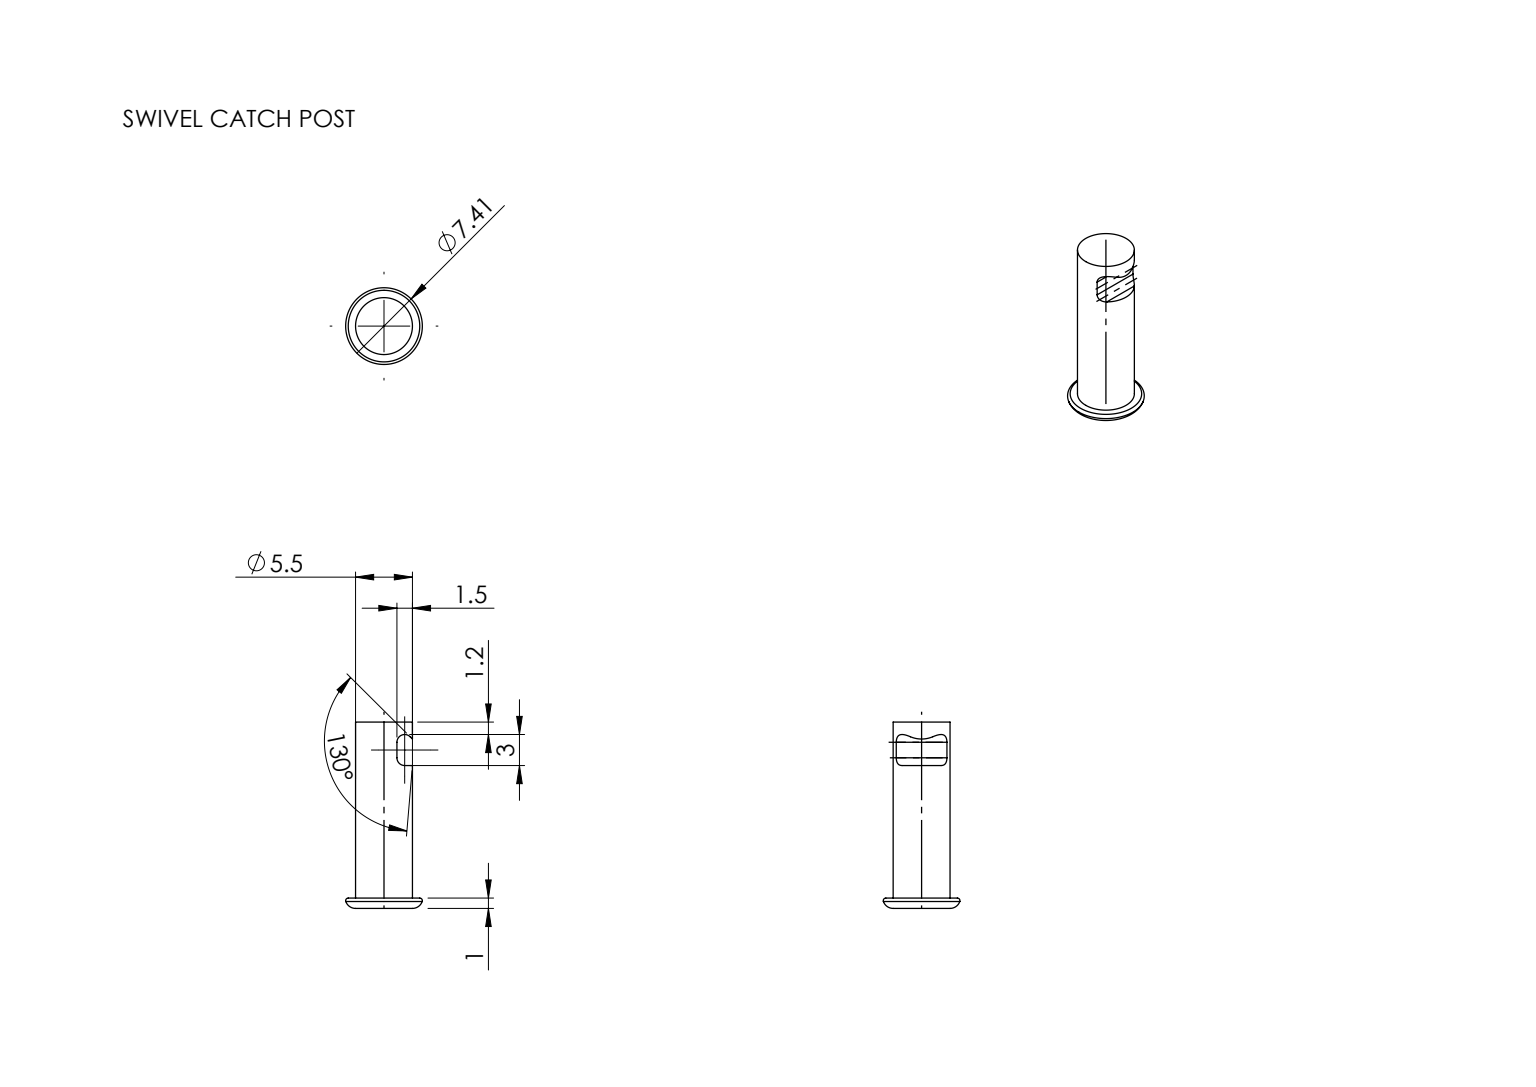
ISO-10303-21;
HEADER;
FILE_DESCRIPTION (('STEP AP214'),
    '1' );
FILE_NAME ('Swivel Catch Post.step',
    '2026-09-30T04:43:20',
    ( '' ),
    ( '' ),
    'SwSTEP 2.0',
    'SolidWorks 2026',
    '' );
FILE_SCHEMA (( 'AUTOMOTIVE_DESIGN' ));
ENDSEC;

DATA;
#106=EDGE_CURVE ( 'NONE', #30303, #19164, #12974, .T. ) ;
#210=LINE ( 'NONE', #17557, #51006 ) ;
#446=ADVANCED_FACE ( 'NONE', ( #32795 ), #44037, .T. ) ;
#717=FACE_OUTER_BOUND ( 'NONE', #44823, .T. ) ;
#818=DIRECTION ( 'NONE',  ( 0.000000000000000000, 1.000000000000000000, 0.000000000000000000 ) ) ;
#927=CARTESIAN_POINT ( 'NONE',  ( -56.75000000000000711, 6.050000000000001599, 2.449489742783185875 ) ) ;
#976=DIRECTION ( 'NONE',  ( 0.000000000000000000, -1.000000000000000000, 0.000000000000000000 ) ) ;
#1009=CIRCLE ( 'NONE', #16413, 2.750000000000001776 ) ;
#1234=CYLINDRICAL_SURFACE ( 'NONE', #12104, 0.7500000000000006661 ) ;
#1569=ORIENTED_EDGE ( 'NONE', *, *, #18264, .F. ) ;
#1965=ORIENTED_EDGE ( 'NONE', *, *, #43779, .F. ) ;
#2198=ORIENTED_EDGE ( 'NONE', *, *, #35348, .F. ) ;
#2411=MANIFOLD_SOLID_BREP ( 'Fillet2', #42168 ) ;
#2610=AXIS2_PLACEMENT_3D ( 'NONE', #34638, #13373, #3697 ) ;
#2848=CARTESIAN_POINT ( 'NONE',  ( -55.47117325737978888, 6.581829179614757663, 1.080525476705103127 ) ) ;
#3278=( NAMED_UNIT ( * ) PLANE_ANGLE_UNIT ( ) SI_UNIT ( $, .RADIAN. ) );
#3473=ADVANCED_FACE ( 'NONE', ( #50960, #8114 ), #12651, .T. ) ;
#3535=VERTEX_POINT ( 'NONE', #55238 ) ;
#3551=( LENGTH_UNIT ( ) NAMED_UNIT ( * ) SI_UNIT ( .MILLI., .METRE. ) );
#3578=CARTESIAN_POINT ( 'NONE',  ( -58.00000000000000711, -9.999999999999998224, 7.102951435054649637E-15 ) ) ;
#3629=CARTESIAN_POINT ( 'NONE',  ( -56.65747392845349850, 6.423369595003239674, -2.400381607668001571 ) ) ;
#3697=DIRECTION ( 'NONE',  ( 1.000000000000000000, 0.000000000000000000, 0.000000000000000000 ) ) ;
#3987=CIRCLE ( 'NONE', #7590, 3.692809041582069352 ) ;
#4028=EDGE_LOOP ( 'NONE', ( #26060, #54634 ) ) ;
#4049=ORIENTED_EDGE ( 'NONE', *, *, #41228, .F. ) ;
#4164=CIRCLE ( 'NONE', #6875, 1.000000000000000000 ) ;
#4191=DIRECTION ( 'NONE',  ( -0.000000000000000000, -0.000000000000000000, 1.000000000000000000 ) ) ;
#4239=FACE_OUTER_BOUND ( 'NONE', #21147, .T. ) ;
#4283=ORIENTED_EDGE ( 'NONE', *, *, #8142, .T. ) ;
#4454=EDGE_CURVE ( 'NONE', #51315, #45422, #36769, .T. ) ;
#4485=CARTESIAN_POINT ( 'NONE',  ( -55.79576865894325977, 6.773981352271770007, -1.647106450292881163 ) ) ;
#4595=DIRECTION ( 'NONE',  ( 0.000000000000000000, 0.000000000000000000, 1.000000000000000000 ) ) ;
#4651=ORIENTED_EDGE ( 'NONE', *, *, #24419, .F. ) ;
#4656=PRODUCT ( 'Swivel Catch Post', 'Swivel Catch Post', '', ( #13009 ) ) ;
#4836=CIRCLE ( 'NONE', #42891, 3.457106781186553235 ) ;
#4927=EDGE_LOOP ( 'NONE', ( #9077, #36170 ) ) ;
#5049=ADVANCED_FACE ( 'NONE', ( #50607 ), #46482, .T. ) ;
#5155=DIRECTION ( 'NONE',  ( -0.000000000000000000, -0.000000000000000000, 1.000000000000000000 ) ) ;
#5423=EDGE_CURVE ( 'NONE', #11807, #36151, #4836, .T. ) ;
#5489=EDGE_LOOP ( 'NONE', ( #39206, #54488 ) ) ;
#5657=TOROIDAL_SURFACE ( 'NONE', #31069, 3.457106781186553235, 0.2500000000000000000 ) ;
#5758=AXIS2_PLACEMENT_3D ( 'NONE', #44985, #31062, #44404 ) ;
#5852=CIRCLE ( 'NONE', #10392, 2.750000000000001776 ) ;
#6089=PRODUCT_DEFINITION_SHAPE ( 'NONE', 'NONE',  #46837 ) ;
#6098=AXIS2_PLACEMENT_3D ( 'NONE', #52656, #26020, #51820 ) ;
#6342=EDGE_CURVE ( 'NONE', #47897, #8966, #3987, .T. ) ;
#6579=CARTESIAN_POINT ( 'NONE',  ( -55.97617513261492661, 6.813462753686547302, 1.872163189751866907 ) ) ;
#6606=EDGE_LOOP ( 'NONE', ( #41022, #15281, #4651, #28201 ) ) ;
#6772=DIRECTION ( 'NONE',  ( 0.000000000000000000, 1.000000000000000000, 0.000000000000000000 ) ) ;
#6829=CARTESIAN_POINT ( 'NONE',  ( -58.00000000000000711, -8.999999999999998224, 2.750000000000013323 ) ) ;
#6875=AXIS2_PLACEMENT_3D ( 'NONE', #10848, #23077, #23368 ) ;
#6928=CARTESIAN_POINT ( 'NONE',  ( -56.00000000000000711, 3.800000000000001599, 1.887458608817694561 ) ) ;
#7213=CARTESIAN_POINT ( 'NONE',  ( -58.00000000000000711, -9.000000000000000000, 7.102951435054649637E-15 ) ) ;
#7257=CARTESIAN_POINT ( 'NONE',  ( -55.47117325737978888, 6.581829179614757663, -1.080525476705088916 ) ) ;
#7453=EDGE_CURVE ( 'NONE', #8966, #47897, #15484, .T. ) ;
#7541=DIRECTION ( 'NONE',  ( 0.000000000000000000, 1.000000000000000000, 0.000000000000000000 ) ) ;
#7590=AXIS2_PLACEMENT_3D ( 'NONE', #8285, #25599, #12827 ) ;
#7684=CARTESIAN_POINT ( 'NONE',  ( -55.47117325737978888, 6.581829179614757663, -1.080525476705088916 ) ) ;
#7794=VECTOR ( 'NONE', #30262, 1000.000000000000000 ) ;
#8114=FACE_OUTER_BOUND ( 'NONE', #6606, .T. ) ;
#8142=EDGE_CURVE ( 'NONE', #45422, #51315, #1009, .T. ) ;
#8210=ORIENTED_EDGE ( 'NONE', *, *, #43779, .T. ) ;
#8223=ORIENTED_EDGE ( 'NONE', *, *, #14640, .T. ) ;
#8264=ORIENTED_EDGE ( 'NONE', *, *, #40320, .F. ) ;
#8285=CARTESIAN_POINT ( 'NONE',  ( -58.00000000000000711, -9.333333333333333925, 7.102951435054649637E-15 ) ) ;
#8429=DIRECTION ( 'NONE',  ( 0.000000000000000000, 1.000000000000000000, 0.000000000000000000 ) ) ;
#8475=DIRECTION ( 'NONE',  ( 0.000000000000000000, 0.000000000000000000, -1.000000000000000000 ) ) ;
#8786=DIRECTION ( 'NONE',  ( -0.000000000000000000, -0.000000000000000000, 1.000000000000000000 ) ) ;
#8966=VERTEX_POINT ( 'NONE', #28731 ) ;
#9077=ORIENTED_EDGE ( 'NONE', *, *, #4454, .F. ) ;
#9245=ORIENTED_EDGE ( 'NONE', *, *, #7453, .T. ) ;
#9495=DIRECTION ( 'NONE',  ( -0.000000000000000000, -0.000000000000000000, 1.000000000000000000 ) ) ;
#9731=AXIS2_PLACEMENT_3D ( 'NONE', #16881, #48351, #13173 ) ;
#9733=CARTESIAN_POINT ( 'NONE',  ( -56.32517369257367079, 3.868430646962533359, -2.183859404458766917 ) ) ;
#9746=APPLICATION_CONTEXT ( 'automotive_design' ) ;
#9865=EDGE_CURVE ( 'NONE', #3535, #28311, #56017, .T. ) ;
#9936=CARTESIAN_POINT ( 'NONE',  ( -58.00000000000000711, -9.000000000000000000, -3.457106781186546129 ) ) ;
#9965=CARTESIAN_POINT ( 'NONE',  ( -58.00000000000000711, -9.000000000000000000, 2.750000000000008438 ) ) ;
#10333=DIRECTION ( 'NONE',  ( -1.000000000000000000, 0.000000000000000000, -0.000000000000000000 ) ) ;
#10392=AXIS2_PLACEMENT_3D ( 'NONE', #34327, #12733, #8475 ) ;
#10736=FACE_OUTER_BOUND ( 'NONE', #5489, .T. ) ;
#10786=ADVANCED_FACE ( 'NONE', ( #10736 ), #24058, .F. ) ;
#10848=CARTESIAN_POINT ( 'NONE',  ( -58.00000000000000711, -8.999999999999998224, -2.749999999999999556 ) ) ;
#10855=CARTESIAN_POINT ( 'NONE',  ( -24.28770178542860947, -24.42559627614718565, -2.749999999999994671 ) ) ;
#10888=CARTESIAN_POINT ( 'NONE',  ( -56.40932156468398517, 3.913516004366899725, 2.245148959471634065 ) ) ;
#10909=DIRECTION ( 'NONE',  ( 0.000000000000000000, -1.000000000000000000, 0.000000000000000000 ) ) ;
#10925=EDGE_CURVE ( 'NONE', #36151, #11807, #55038, .T. ) ;
#11019=ORIENTED_EDGE ( 'NONE', *, *, #7453, .F. ) ;
#11426=ADVANCED_FACE ( 'NONE', ( #56060 ), #17711, .T. ) ;
#11522=DIRECTION ( 'NONE',  ( 0.000000000000000000, -1.000000000000000000, 0.000000000000000000 ) ) ;
#11576=DIRECTION ( 'NONE',  ( -0.000000000000000000, 1.000000000000000000, -0.000000000000000000 ) ) ;
#11607=EDGE_CURVE ( 'NONE', #45422, #39433, #35883, .T. ) ;
#11689=ORIENTED_EDGE ( 'NONE', *, *, #26993, .T. ) ;
#11777=ORIENTED_EDGE ( 'NONE', *, *, #41228, .T. ) ;
#11807=VERTEX_POINT ( 'NONE', #9936 ) ;
#11982=CARTESIAN_POINT ( 'NONE',  ( -56.75000000000000711, -9.000000000000000000, -2.449489742783172108 ) ) ;
#12104=AXIS2_PLACEMENT_3D ( 'NONE', #44676, #9495, #18868 ) ;
#12280=ORIENTED_EDGE ( 'NONE', *, *, #21641, .F. ) ;
#12377=FILL_AREA_STYLE ('',( #29957 ) ) ;
#12476=DIRECTION ( 'NONE',  ( 1.000000000000000000, 0.000000000000000000, 0.000000000000000000 ) ) ;
#12488=AXIS2_PLACEMENT_3D ( 'NONE', #3578, #25186, #41901 ) ;
#12651=CYLINDRICAL_SURFACE ( 'NONE', #41209, 2.750000000000001776 ) ;
#12705=ADVANCED_FACE ( 'NONE', ( #52110 ), #55979, .T. ) ;
#12717=CARTESIAN_POINT ( 'NONE',  ( -56.40927410319390134, 6.683688692736960313, -2.245073662639579304 ) ) ;
#12726=SHAPE_DEFINITION_REPRESENTATION ( #6089, #55389 ) ;
#12733=DIRECTION ( 'NONE',  ( -0.000000000000000000, 1.000000000000000000, -0.000000000000000000 ) ) ;
#12827=DIRECTION ( 'NONE',  ( 0.000000000000000000, 0.000000000000000000, 1.000000000000000000 ) ) ;
#12917=AXIS2_PLACEMENT_3D ( 'NONE', #7213, #10909, #24263 ) ;
#12974=LINE ( 'NONE', #47317, #16801 ) ;
#13009=PRODUCT_CONTEXT ( 'NONE', #9746, 'mechanical' ) ;
#13173=DIRECTION ( 'NONE',  ( 0.000000000000000000, -0.000000000000000000, -1.000000000000000000 ) ) ;
#13373=DIRECTION ( 'NONE',  ( 0.000000000000000000, 0.000000000000000000, 1.000000000000000000 ) ) ;
#13398=CARTESIAN_POINT ( 'NONE',  ( -56.75000000000000711, 6.050000000000001599, -2.749999999999994671 ) ) ;
#13741=FACE_OUTER_BOUND ( 'NONE', #52868, .T. ) ;
#13747=EDGE_LOOP ( 'NONE', ( #25210, #8223, #11019, #4049 ) ) ;
#13765=CARTESIAN_POINT ( 'NONE',  ( -58.00000000000000711, -9.250000000000000000, 7.102951435054649637E-15 ) ) ;
#13893=DIRECTION ( 'NONE',  ( 0.000000000000000000, 1.000000000000000000, 0.000000000000000000 ) ) ;
#14023=CARTESIAN_POINT ( 'NONE',  ( -58.00000000000000711, -9.000000000000000000, 7.102951435054649637E-15 ) ) ;
#14277=CARTESIAN_POINT ( 'NONE',  ( -56.75000000000000711, 4.550000000000001599, -2.449489742783172108 ) ) ;
#14309=CARTESIAN_POINT ( 'NONE',  ( -58.00000000000000711, -9.000000000000000000, -2.749999999999994671 ) ) ;
#14387=EDGE_CURVE ( 'NONE', #8966, #28311, #4164, .T. ) ;
#14529=CARTESIAN_POINT ( 'NONE',  ( -56.75000000000000711, 4.436543092327784876, -2.449489742783172996 ) ) ;
#14559=DIRECTION ( 'NONE',  ( 0.7091055728196409280, -0.7051023234936394379, 0.000000000000000000 ) ) ;
#14640=EDGE_CURVE ( 'NONE', #36151, #47897, #36794, .T. ) ;
#14755=CIRCLE ( 'NONE', #43758, 2.750000000000001776 ) ;
#14829=CARTESIAN_POINT ( 'NONE',  ( -56.40853634832227925, 6.684187361877747868, 2.244562702769390405 ) ) ;
#14841=FACE_OUTER_BOUND ( 'NONE', #33369, .T. ) ;
#15281=ORIENTED_EDGE ( 'NONE', *, *, #11607, .T. ) ;
#15484=CIRCLE ( 'NONE', #38148, 3.692809041582069352 ) ;
#15630=CARTESIAN_POINT ( 'NONE',  ( -58.00000000000000711, -9.999999999999998224, 7.102951435054649637E-15 ) ) ;
#15739=CIRCLE ( 'NONE', #47489, 1.000000000000000000 ) ;
#15804=DIRECTION ( 'NONE',  ( 0.000000000000000000, 0.000000000000000000, -1.000000000000000000 ) ) ;
#15899=AXIS2_PLACEMENT_3D ( 'NONE', #36805, #11522, #41039 ) ;
#15965=AXIS2_PLACEMENT_3D ( 'NONE', #30563, #52950, #39053 ) ;
#16203=CARTESIAN_POINT ( 'NONE',  ( -55.17209868701984732, 6.284443032133043339, -0.3805810627426228776 ) ) ;
#16235=COLOUR_RGB ( '', 0.09019608, 0.27058824, 0.51372549) ;
#16258=APPLICATION_CONTEXT ( 'automotive_design' ) ;
#16298=CARTESIAN_POINT ( 'NONE',  ( -58.00000000000000711, 8.000000000000000000, 7.102951435054649637E-15 ) ) ;
#16413=AXIS2_PLACEMENT_3D ( 'NONE', #49665, #6772, #45126 ) ;
#16474=SURFACE_STYLE_FILL_AREA ( #34949 ) ;
#16801=VECTOR ( 'NONE', #4191, 1000.000000000000000 ) ;
#16831=ADVANCED_FACE ( 'NONE', ( #27358 ), #36184, .F. ) ;
#16834=CARTESIAN_POINT ( 'NONE',  ( -58.00000000000000711, 8.000000000000000000, 7.102951435054649637E-15 ) ) ;
#16881=CARTESIAN_POINT ( 'NONE',  ( -58.00000000000000711, -9.999999999999998224, 7.102951435054649637E-15 ) ) ;
#17063=( NAMED_UNIT ( * ) SI_UNIT ( $, .STERADIAN. ) SOLID_ANGLE_UNIT ( ) );
#17413=DIRECTION ( 'NONE',  ( 0.000000000000000000, 0.000000000000000000, 1.000000000000000000 ) ) ;
#17534=CARTESIAN_POINT ( 'NONE',  ( -56.60431429388330571, 6.503145704592061982, -2.370631253071207922 ) ) ;
#17557=CARTESIAN_POINT ( 'NONE',  ( -56.00000000000000711, 3.800000000000001599, -2.749999999999994671 ) ) ;
#17640=DIRECTION ( 'NONE',  ( 0.000000000000000000, 1.000000000000000000, 0.000000000000000000 ) ) ;
#17664=DIRECTION ( 'NONE',  ( 0.000000000000000000, -1.000000000000000000, 0.000000000000000000 ) ) ;
#17711=PLANE ( 'NONE',  #9731 ) ;
#18264=EDGE_CURVE ( 'NONE', #48789, #29854, #42161, .T. ) ;
#18503=CARTESIAN_POINT ( 'NONE',  ( -56.15823370927599001, 3.811598478745688023, -2.045038383219965894 ) ) ;
#18868=DIRECTION ( 'NONE',  ( 1.000000000000000000, 0.000000000000000000, 0.000000000000000000 ) ) ;
#19164=VERTEX_POINT ( 'NONE', #31350 ) ;
#19352=CARTESIAN_POINT ( 'NONE',  ( -55.84725198092744591, 6.793269954351565332, 1.721684726214605998 ) ) ;
#19364=DIRECTION ( 'NONE',  ( -0.7051023234936394379, -0.7091055728196409280, 0.000000000000000000 ) ) ;
#20049=CARTESIAN_POINT ( 'NONE',  ( -58.00000000000000711, -9.000000000000000000, 7.102951435054649637E-15 ) ) ;
#20178=CARTESIAN_POINT ( 'NONE',  ( -55.54283117668188652, 6.653082554758466216, 1.248231344413326394 ) ) ;
#20257=FACE_OUTER_BOUND ( 'NONE', #4028, .T. ) ;
#20315=CARTESIAN_POINT ( 'NONE',  ( -58.00000000000000711, 8.000000000000000000, 7.102951435054649637E-15 ) ) ;
#20494=VERTEX_POINT ( 'NONE', #39393 ) ;
#20778=STYLED_ITEM ( 'NONE', ( #47425 ), #49640 ) ;
#20796=FACE_OUTER_BOUND ( 'NONE', #42057, .T. ) ;
#20913=VERTEX_POINT ( 'NONE', #35839 ) ;
#21012=SHAPE_REPRESENTATION_RELATIONSHIP ( 'NONE' , 'NONE' ,  #55389, #49640 ) ;
#21116=LINE ( 'NONE', #35057, #30207 ) ;
#21147=EDGE_LOOP ( 'NONE', ( #31251, #25114, #24414, #22015 ) ) ;
#21202=ORIENTED_EDGE ( 'NONE', *, *, #14387, .F. ) ;
#21641=EDGE_CURVE ( 'NONE', #40359, #30303, #40783, .T. ) ;
#21701=DIRECTION ( 'NONE',  ( 0.000000000000000000, 1.000000000000000000, 0.000000000000000000 ) ) ;
#21726=PRODUCT_DEFINITION_FORMATION_WITH_SPECIFIED_SOURCE ( 'ANY', '', #4656, .NOT_KNOWN. ) ;
#21740=CYLINDRICAL_SURFACE ( 'NONE', #15965, 2.750000000000001776 ) ;
#21794=CARTESIAN_POINT ( 'NONE',  ( -56.75000000000000711, 6.050000000000001599, -2.449489742783172108 ) ) ;
#21847=EDGE_CURVE ( 'NONE', #39433, #20494, #14755, .T. ) ;
#22015=ORIENTED_EDGE ( 'NONE', *, *, #23716, .F. ) ;
#22053=VECTOR ( 'NONE', #17640, 1000.000000000000000 ) ;
#22431=EDGE_LOOP ( 'NONE', ( #30912, #42795, #39124, #36013, #33556, #12280, #2198, #1569 ) ) ;
#23015=ORIENTED_EDGE ( 'NONE', *, *, #31360, .T. ) ;
#23077=DIRECTION ( 'NONE',  ( -1.000000000000000000, -0.000000000000000000, -0.000000000000000000 ) ) ;
#23368=DIRECTION ( 'NONE',  ( 0.000000000000000000, 0.000000000000000000, 1.000000000000000000 ) ) ;
#23492=ADVANCED_FACE ( 'NONE', ( #14841 ), #53721, .T. ) ;
#23716=EDGE_CURVE ( 'NONE', #40359, #47613, #48273, .T. ) ;
#23946=CARTESIAN_POINT ( 'NONE',  ( -56.07727432805427981, 3.800000000000001155, 1.969340487120371019 ) ) ;
#24058=PLANE ( 'NONE',  #46848 ) ;
#24195=CARTESIAN_POINT ( 'NONE',  ( -56.65661634607675978, 6.425189153618619642, 2.399912804366261643 ) ) ;
#24263=DIRECTION ( 'NONE',  ( 0.000000000000000000, -0.000000000000000000, -1.000000000000000000 ) ) ;
#24409=DIRECTION ( 'NONE',  ( 1.000000000000000000, 0.000000000000000000, -1.224646799147353207E-16 ) ) ;
#24414=ORIENTED_EDGE ( 'NONE', *, *, #39666, .T. ) ;
#24419=EDGE_CURVE ( 'NONE', #20494, #39433, #42009, .T. ) ;
#24686=EDGE_LOOP ( 'NONE', ( #39980, #48644, #11777, #45574 ) ) ;
#25090=CARTESIAN_POINT ( 'NONE',  ( -56.75000000000001421, 4.436683557093994423, 2.449489742783185875 ) ) ;
#25114=ORIENTED_EDGE ( 'NONE', *, *, #106, .T. ) ;
#25186=DIRECTION ( 'NONE',  ( 0.000000000000000000, -1.000000000000000000, 0.000000000000000000 ) ) ;
#25210=ORIENTED_EDGE ( 'NONE', *, *, #10925, .F. ) ;
#25232=CARTESIAN_POINT ( 'NONE',  ( -56.75000000000001421, 6.148917331397711017, -2.449489742783171664 ) ) ;
#25420=DIRECTION ( 'NONE',  ( 0.000000000000000000, 0.000000000000000000, 1.000000000000000000 ) ) ;
#25488=CARTESIAN_POINT ( 'NONE',  ( -55.63255288014424593, 6.714018351055213607, -1.412117554830255362 ) ) ;
#25599=DIRECTION ( 'NONE',  ( 0.000000000000000000, -1.000000000000000000, 0.000000000000000000 ) ) ;
#25865=( NAMED_UNIT ( * ) PLANE_ANGLE_UNIT ( ) SI_UNIT ( $, .RADIAN. ) );
#25936=AXIS2_PLACEMENT_3D ( 'NONE', #34392, #30421, #51973 ) ;
#26020=DIRECTION ( 'NONE',  ( 0.000000000000000000, -1.000000000000000000, 0.000000000000000000 ) ) ;
#26060=ORIENTED_EDGE ( 'NONE', *, *, #5423, .T. ) ;
#26080=CARTESIAN_POINT ( 'NONE',  ( -56.26447305843585411, 6.756484714774108724, -2.135113782577493513 ) ) ;
#26136=CARTESIAN_POINT ( 'NONE',  ( -55.17209868701984732, 6.284443032133044227, 0.3805810627426376991 ) ) ;
#26396=( LENGTH_UNIT ( ) NAMED_UNIT ( * ) SI_UNIT ( .MILLI., .METRE. ) );
#26610=VECTOR ( 'NONE', #34165, 1000.000000000000000 ) ;
#26938=CARTESIAN_POINT ( 'NONE',  ( -56.75000000000000711, 6.050000000000001599, -2.449489742783172108 ) ) ;
#26993=EDGE_CURVE ( 'NONE', #50717, #20913, #34858, .T. ) ;
#27040=CARTESIAN_POINT ( 'NONE',  ( -56.40918267430362221, 3.913378331250040087, -2.245061400351528569 ) ) ;
#27358=FACE_OUTER_BOUND ( 'NONE', #28823, .T. ) ;
#27706=CIRCLE ( 'NONE', #47728, 2.750000000000006217 ) ;
#28043=CARTESIAN_POINT ( 'NONE',  ( 0.000000000000000000, 3.800000000000002043, -2.749999999999994671 ) ) ;
#28156=CARTESIAN_POINT ( 'NONE',  ( -56.60439204777216560, 6.503221467314357795, 2.370703063681847134 ) ) ;
#28201=ORIENTED_EDGE ( 'NONE', *, *, #47935, .F. ) ;
#28203=CARTESIAN_POINT ( 'NONE',  ( -56.32449333261072155, 3.868143273367939727, 2.183322036886178097 ) ) ;
#28311=VERTEX_POINT ( 'NONE', #36142 ) ;
#28504=PLANE ( 'NONE',  #12917 ) ;
#28731=CARTESIAN_POINT ( 'NONE',  ( -58.00000000000000711, -9.333333333333333925, -3.692809041582062246 ) ) ;
#28823=EDGE_LOOP ( 'NONE', ( #32458, #1965, #52851, #40119 ) ) ;
#29107=PRODUCT_DEFINITION_CONTEXT ( 'detailed design', #16258, 'design' ) ;
#29112=CARTESIAN_POINT ( 'NONE',  ( -58.00000000000000711, -9.000000000000000000, 7.102951435054649637E-15 ) ) ;
#29396=( NAMED_UNIT ( * ) SI_UNIT ( $, .STERADIAN. ) SOLID_ANGLE_UNIT ( ) );
#29573=( NAMED_UNIT ( * ) SI_UNIT ( $, .STERADIAN. ) SOLID_ANGLE_UNIT ( ) );
#29854=VERTEX_POINT ( 'NONE', #44099 ) ;
#29957=FILL_AREA_STYLE_COLOUR ( '', #48271 ) ;
#30036=CARTESIAN_POINT ( 'NONE',  ( -56.19068569781688893, 6.778861748851165103, -2.073212483771301073 ) ) ;
#30183=EDGE_LOOP ( 'NONE', ( #23015, #48028 ) ) ;
#30207=VECTOR ( 'NONE', #47527, 1000.000000000000000 ) ;
#30262=DIRECTION ( 'NONE',  ( -0.000000000000000000, -0.000000000000000000, 1.000000000000000000 ) ) ;
#30303=VERTEX_POINT ( 'NONE', #7257 ) ;
#30404=SURFACE_STYLE_USAGE ( .BOTH. , #51121 ) ;
#30421=DIRECTION ( 'NONE',  ( 1.000000000000000000, 0.000000000000000000, -1.224646799147353207E-16 ) ) ;
#30563=CARTESIAN_POINT ( 'NONE',  ( -58.00000000000000711, -9.000000000000000000, 7.102951435054649637E-15 ) ) ;
#30912=ORIENTED_EDGE ( 'NONE', *, *, #48807, .F. ) ;
#31062=DIRECTION ( 'NONE',  ( -1.000000000000000000, -0.000000000000000000, -0.000000000000000000 ) ) ;
#31069=AXIS2_PLACEMENT_3D ( 'NONE', #13765, #976, #31932 ) ;
#31251=ORIENTED_EDGE ( 'NONE', *, *, #21641, .T. ) ;
#31294=CARTESIAN_POINT ( 'NONE',  ( -56.07732056155856526, 3.800000000000001155, -1.969389477338281624 ) ) ;
#31350=CARTESIAN_POINT ( 'NONE',  ( -55.47117325737978888, 6.581829179614757663, 1.080525476705103127 ) ) ;
#31360=EDGE_CURVE ( 'NONE', #28311, #3535, #27706, .T. ) ;
#31932=DIRECTION ( 'NONE',  ( 0.000000000000000000, 0.000000000000000000, -1.000000000000000000 ) ) ;
#31960=STYLED_ITEM ( 'NONE', ( #37636 ), #2411 ) ;
#32458=ORIENTED_EDGE ( 'NONE', *, *, #47523, .T. ) ;
#32493=CARTESIAN_POINT ( 'NONE',  ( -56.63016842841614817, 4.129031330634377994, 2.385144069838411873 ) ) ;
#32510=FACE_BOUND ( 'NONE', #4927, .T. ) ;
#32795=FACE_OUTER_BOUND ( 'NONE', #53183, .T. ) ;
#32979=CARTESIAN_POINT ( 'NONE',  ( -56.47915852223218280, 6.634043282999704694, 2.292377755077263934 ) ) ;
#33369=EDGE_LOOP ( 'NONE', ( #42457, #56083 ) ) ;
#33556=ORIENTED_EDGE ( 'NONE', *, *, #36953, .T. ) ;
#33666=( BOUNDED_CURVE ( )  B_SPLINE_CURVE ( 3, ( #42336, #26136, #16203, #7684 ),
 .UNSPECIFIED., .F., .F. ) 
 B_SPLINE_CURVE_WITH_KNOTS ( ( 4, 4 ),
 ( 2.737789607505189515, 3.545395699674396717 ),
 .UNSPECIFIED. ) 
 CURVE ( )  GEOMETRIC_REPRESENTATION_ITEM ( )  RATIONAL_B_SPLINE_CURVE ( ( 1.000000000000000000, 0.9463822406352063732, 0.9463822406352063732, 1.000000000000000000 ) ) 
 REPRESENTATION_ITEM ( '' )  );
#33805=( NAMED_UNIT ( * ) PLANE_ANGLE_UNIT ( ) SI_UNIT ( $, .RADIAN. ) );
#34165=DIRECTION ( 'NONE',  ( 0.000000000000000000, 1.000000000000000000, 0.000000000000000000 ) ) ;
#34327=CARTESIAN_POINT ( 'NONE',  ( -58.00000000000000711, 3.800000000000002931, 7.102951435054649637E-15 ) ) ;
#34340=EDGE_CURVE ( 'NONE', #47897, #3535, #15739, .T. ) ;
#34392=CARTESIAN_POINT ( 'NONE',  ( -58.00000000000000711, -9.250000000000000000, 3.457106781186559896 ) ) ;
#34508=LINE ( 'NONE', #51821, #7794 ) ;
#34534=ORIENTED_EDGE ( 'NONE', *, *, #6342, .T. ) ;
#34638=CARTESIAN_POINT ( 'NONE',  ( 0.000000000000000000, 0.000000000000000000, 0.000000000000000000 ) ) ;
#34693=CARTESIAN_POINT ( 'NONE',  ( -58.00000000000000711, -9.333333333333333925, 7.102951435054649637E-15 ) ) ;
#34858=B_SPLINE_CURVE_WITH_KNOTS ( 'NONE', 3,
 ( #54327, #25090, #37278, #32493, #49795, #10888, #28203, #45512, #23946, #6928 ),
 .UNSPECIFIED., .F., .F.,
 ( 4, 2, 2, 2, 4 ),
 ( 0.000000000000000000, 0.0003349897808261797561, 0.0006699795616523595123, 0.001004969342478539323, 0.001339959123304719025 ),
 .UNSPECIFIED. ) ;
#34949=FILL_AREA_STYLE ('',( #56227 ) ) ;
#35057=CARTESIAN_POINT ( 'NONE',  ( -56.75000000000000711, -9.000000000000000000, 2.449489742783185875 ) ) ;
#35308=MECHANICAL_DESIGN_GEOMETRIC_PRESENTATION_REPRESENTATION('',(#20778),#52518);
#35343=ADVANCED_FACE ( 'NONE', ( #20796 ), #55718, .T. ) ;
#35348=EDGE_CURVE ( 'NONE', #29854, #40359, #55426, .T. ) ;
#35362=FACE_OUTER_BOUND ( 'NONE', #13747, .T. ) ;
#35660=AXIS2_PLACEMENT_3D ( 'NONE', #16834, #818, #48227 ) ;
#35738=AXIS2_PLACEMENT_3D ( 'NONE', #50314, #41530, #40952 ) ;
#35839=CARTESIAN_POINT ( 'NONE',  ( -56.00000000000000711, 3.800000000000001599, 1.887458608817694561 ) ) ;
#35846=CARTESIAN_POINT ( 'NONE',  ( -56.56312404709360919, 4.044422194259722936, -2.346569400431943730 ) ) ;
#35883=LINE ( 'NONE', #14309, #54960 ) ;
#36013=ORIENTED_EDGE ( 'NONE', *, *, #39666, .F. ) ;
#36142=CARTESIAN_POINT ( 'NONE',  ( -58.00000000000000711, -9.999999999999998224, -2.749999999999999556 ) ) ;
#36151=VERTEX_POINT ( 'NONE', #52097 ) ;
#36170=ORIENTED_EDGE ( 'NONE', *, *, #8142, .F. ) ;
#36184=PLANE ( 'NONE',  #54068 ) ;
#36608=AXIS2_PLACEMENT_3D ( 'NONE', #55322, #47090, #12476 ) ;
#36691=CARTESIAN_POINT ( 'NONE',  ( -56.75000000000000711, 6.050000000000001599, 2.449489742783185875 ) ) ;
#36769=CIRCLE ( 'NONE', #42226, 2.750000000000001776 ) ;
#36794=CIRCLE ( 'NONE', #25936, 0.2499999999999997780 ) ;
#36805=CARTESIAN_POINT ( 'NONE',  ( -58.00000000000000711, -8.999999999999998224, 7.102951435054649637E-15 ) ) ;
#36953=EDGE_CURVE ( 'NONE', #19164, #30303, #33666, .T. ) ;
#37092=UNCERTAINTY_MEASURE_WITH_UNIT (LENGTH_MEASURE( 1.000000000000000082E-05 ), #3551, 'distance_accuracy_value', 'NONE');
#37227=CARTESIAN_POINT ( 'NONE',  ( -56.73047118268372202, 6.245764598936942136, 2.439786402985463898 ) ) ;
#37278=CARTESIAN_POINT ( 'NONE',  ( -56.72378334990722237, 4.325356880459150233, 2.436518382942996830 ) ) ;
#37384=DIRECTION ( 'NONE',  ( 0.000000000000000000, 0.000000000000000000, -1.000000000000000000 ) ) ;
#37515=CARTESIAN_POINT ( 'NONE',  ( -56.19049806081029175, 6.779003593249485426, 2.073111974254101320 ) ) ;
#37636=PRESENTATION_STYLE_ASSIGNMENT (( #42463 ) ) ;
#37650=DIRECTION ( 'NONE',  ( 0.000000000000000000, 1.000000000000000000, 0.000000000000000000 ) ) ;
#38148=AXIS2_PLACEMENT_3D ( 'NONE', #34693, #17664, #4595 ) ;
#38259=CARTESIAN_POINT ( 'NONE',  ( -56.48048524421252381, 6.632812770515467804, -2.293230480183058528 ) ) ;
#38371=LINE ( 'NONE', #43224, #22053 ) ;
#38417=AXIS2_PLACEMENT_3D ( 'NONE', #16298, #21701, #17413 ) ;
#38910=( GEOMETRIC_REPRESENTATION_CONTEXT ( 3 ) GLOBAL_UNCERTAINTY_ASSIGNED_CONTEXT ( ( #51263 ) ) GLOBAL_UNIT_ASSIGNED_CONTEXT ( ( #26396, #33805, #17063 ) ) REPRESENTATION_CONTEXT ( 'NONE', 'WORKASPACE' ) );
#39053=DIRECTION ( 'NONE',  ( 0.000000000000000000, 0.000000000000000000, 1.000000000000000000 ) ) ;
#39110=CARTESIAN_POINT ( 'NONE',  ( -55.47117325737978888, 6.581829179614757663, -1.080525476705088916 ) ) ;
#39124=ORIENTED_EDGE ( 'NONE', *, *, #47523, .F. ) ;
#39206=ORIENTED_EDGE ( 'NONE', *, *, #40320, .T. ) ;
#39291=ADVANCED_FACE ( 'NONE', ( #35362 ), #5657, .T. ) ;
#39334=ADVANCED_FACE ( 'NONE', ( #20257, #32510 ), #28504, .F. ) ;
#39393=CARTESIAN_POINT ( 'NONE',  ( -58.00000000000000711, 8.000000000000000000, 2.750000000000008438 ) ) ;
#39433=VERTEX_POINT ( 'NONE', #45532 ) ;
#39595=ORIENTED_EDGE ( 'NONE', *, *, #34340, .T. ) ;
#39666=EDGE_CURVE ( 'NONE', #19164, #47613, #50163, .T. ) ;
#39980=ORIENTED_EDGE ( 'NONE', *, *, #14640, .F. ) ;
#40119=ORIENTED_EDGE ( 'NONE', *, *, #23716, .T. ) ;
#40191=ORIENTED_EDGE ( 'NONE', *, *, #18264, .T. ) ;
#40320=EDGE_CURVE ( 'NONE', #48789, #20913, #210, .T. ) ;
#40359=VERTEX_POINT ( 'NONE', #26938 ) ;
#40519=ORIENTED_EDGE ( 'NONE', *, *, #47935, .T. ) ;
#40664=CARTESIAN_POINT ( 'NONE',  ( -56.62967144059850000, 4.128180327486781209, -2.384865143139781374 ) ) ;
#40710=DIRECTION ( 'NONE',  ( 0.000000000000000000, 0.000000000000000000, 1.000000000000000000 ) ) ;
#40783=B_SPLINE_CURVE_WITH_KNOTS ( 'NONE', 3,
 ( #21794, #25232, #42538, #3629, #17534, #38259, #12717, #26080, #30036, #55583, #51346, #43389, #4485, #25488, #42796, #39110 ),
 .UNSPECIFIED., .F., .F.,
 ( 4, 2, 2, 2, 2, 2, 2, 4 ),
 ( 0.000000000000000000, 0.0002924226556627319796, 0.0005848453113254639592, 0.0008772679669881960473, 0.001169690622650927918, 0.001462113278313660440, 0.001754535933976393179, 0.002339381245301844995 ),
 .UNSPECIFIED. ) ;
#40952=DIRECTION ( 'NONE',  ( 0.000000000000000000, 0.000000000000000000, -1.000000000000000000 ) ) ;
#41022=ORIENTED_EDGE ( 'NONE', *, *, #4454, .T. ) ;
#41039=DIRECTION ( 'NONE',  ( 0.000000000000000000, 0.000000000000000000, -1.000000000000000000 ) ) ;
#41194=ADVANCED_FACE ( 'NONE', ( #13741 ), #1234, .F. ) ;
#41209=AXIS2_PLACEMENT_3D ( 'NONE', #29112, #37650, #25420 ) ;
#41221=CARTESIAN_POINT ( 'NONE',  ( -55.63114022126601554, 6.713117369705148718, 1.409618983554703719 ) ) ;
#41228=EDGE_CURVE ( 'NONE', #11807, #8966, #48386, .T. ) ;
#41511=CARTESIAN_POINT ( 'NONE',  ( -56.75000000000001421, 6.149180203093333574, 2.449489742783260038 ) ) ;
#41530=DIRECTION ( 'NONE',  ( 0.000000000000000000, -1.000000000000000000, 0.000000000000000000 ) ) ;
#41749=DIRECTION ( 'NONE',  ( 0.000000000000000000, 0.000000000000000000, -1.000000000000000000 ) ) ;
#41901=DIRECTION ( 'NONE',  ( 0.000000000000000000, 0.000000000000000000, -1.000000000000000000 ) ) ;
#42009=CIRCLE ( 'NONE', #38417, 2.750000000000001776 ) ;
#42057=EDGE_LOOP ( 'NONE', ( #54737, #55252 ) ) ;
#42147=CARTESIAN_POINT ( 'NONE',  ( -56.75000000000000711, 4.550000000000001599, 2.449489742783185875 ) ) ;
#42161=B_SPLINE_CURVE_WITH_KNOTS ( 'NONE', 3,
 ( #48622, #31294, #18503, #9733, #27040, #35846, #40664, #53169, #14529, #14277 ),
 .UNSPECIFIED., .F., .F.,
 ( 4, 2, 2, 2, 4 ),
 ( 0.000000000000000000, 0.0003339141718491685099, 0.0006678283436983370198, 0.001001742515547505638, 0.001335656687396674040 ),
 .UNSPECIFIED. ) ;
#42168=CLOSED_SHELL ( 'NONE', ( #39291, #12705, #3473, #43879, #35343, #10786, #41194, #16831, #48753, #23492, #11426, #39334, #446, #5049 ) ) ;
#42172=SURFACE_STYLE_FILL_AREA ( #12377 ) ;
#42188=DIRECTION ( 'NONE',  ( 0.000000000000000000, 0.000000000000000000, 1.000000000000000000 ) ) ;
#42226=AXIS2_PLACEMENT_3D ( 'NONE', #14023, #8429, #40710 ) ;
#42336=CARTESIAN_POINT ( 'NONE',  ( -55.47117325737978888, 6.581829179614757663, 1.080525476705103127 ) ) ;
#42457=ORIENTED_EDGE ( 'NONE', *, *, #106, .F. ) ;
#42463=SURFACE_STYLE_USAGE ( .BOTH. , #46714 ) ;
#42538=CARTESIAN_POINT ( 'NONE',  ( -56.73021393513262467, 6.246123507023290777, -2.439641667270313619 ) ) ;
#42795=ORIENTED_EDGE ( 'NONE', *, *, #26993, .F. ) ;
#42796=CARTESIAN_POINT ( 'NONE',  ( -55.54282512360118318, 6.653076535853754692, -1.248217177980195380 ) ) ;
#42891=AXIS2_PLACEMENT_3D ( 'NONE', #51317, #11576, #37384 ) ;
#43224=CARTESIAN_POINT ( 'NONE',  ( -58.00000000000000711, -9.000000000000000000, 2.750000000000008438 ) ) ;
#43281=ORIENTED_EDGE ( 'NONE', *, *, #11607, .F. ) ;
#43389=CARTESIAN_POINT ( 'NONE',  ( -55.85443948382626900, 6.788488266608555755, -1.722920386167723583 ) ) ;
#43475=ORIENTED_EDGE ( 'NONE', *, *, #34340, .F. ) ;
#43736=MECHANICAL_DESIGN_GEOMETRIC_PRESENTATION_REPRESENTATION('',(#31960),#50984);
#43758=AXIS2_PLACEMENT_3D ( 'NONE', #20315, #7541, #42188 ) ;
#43779=EDGE_CURVE ( 'NONE', #29854, #50717, #34508, .T. ) ;
#43879=ADVANCED_FACE ( 'NONE', ( #717 ), #21740, .T. ) ;
#44037=TOROIDAL_SURFACE ( 'NONE', #15899, 2.750000000000006217, 1.000000000000000000 ) ;
#44099=CARTESIAN_POINT ( 'NONE',  ( -56.75000000000000711, 4.550000000000001599, -2.449489742783172108 ) ) ;
#44404=DIRECTION ( 'NONE',  ( 0.000000000000000000, 0.000000000000000000, 1.000000000000000000 ) ) ;
#44676=CARTESIAN_POINT ( 'NONE',  ( -56.00000000000000711, 4.550000000000001599, -2.749999999999994671 ) ) ;
#44735=ORIENTED_EDGE ( 'NONE', *, *, #14387, .T. ) ;
#44823=EDGE_LOOP ( 'NONE', ( #43281, #4283, #40519, #50145 ) ) ;
#44985=CARTESIAN_POINT ( 'NONE',  ( -58.00000000000000711, -9.250000000000000000, -3.457106781186546129 ) ) ;
#45126=DIRECTION ( 'NONE',  ( 0.000000000000000000, 0.000000000000000000, 1.000000000000000000 ) ) ;
#45280=ORIENTED_EDGE ( 'NONE', *, *, #31360, .F. ) ;
#45347=DIRECTION ( 'NONE',  ( 0.000000000000000000, -0.000000000000000000, -1.000000000000000000 ) ) ;
#45422=VERTEX_POINT ( 'NONE', #55068 ) ;
#45512=CARTESIAN_POINT ( 'NONE',  ( -56.15805904048855979, 3.811595058059581209, 2.044864594757502818 ) ) ;
#45532=CARTESIAN_POINT ( 'NONE',  ( -58.00000000000000711, 8.000000000000000000, -2.749999999999994671 ) ) ;
#45574=ORIENTED_EDGE ( 'NONE', *, *, #6342, .F. ) ;
#46014=EDGE_LOOP ( 'NONE', ( #9245, #39595, #45280, #21202 ) ) ;
#46482=TOROIDAL_SURFACE ( 'NONE', #35738, 3.457106781186553235, 0.2500000000000000000 ) ;
#46714=SURFACE_SIDE_STYLE ('',( #42172 ) ) ;
#46837=PRODUCT_DEFINITION ( 'UNKNOWN', '', #21726, #29107 ) ;
#46848=AXIS2_PLACEMENT_3D ( 'NONE', #28043, #54166, #45347 ) ;
#47090=DIRECTION ( 'NONE',  ( -0.000000000000000000, -0.000000000000000000, 1.000000000000000000 ) ) ;
#47164=CARTESIAN_POINT ( 'NONE',  ( -58.00000000000000711, -9.333333333333333925, 3.692809041582076013 ) ) ;
#47317=CARTESIAN_POINT ( 'NONE',  ( -55.47117325737978888, 6.581829179614757663, -2.749999999999994671 ) ) ;
#47425=PRESENTATION_STYLE_ASSIGNMENT (( #30404 ) ) ;
#47489=AXIS2_PLACEMENT_3D ( 'NONE', #6829, #24409, #55630 ) ;
#47523=EDGE_CURVE ( 'NONE', #47613, #50717, #21116, .T. ) ;
#47527=DIRECTION ( 'NONE',  ( -0.000000000000000000, -1.000000000000000000, -0.000000000000000000 ) ) ;
#47613=VERTEX_POINT ( 'NONE', #927 ) ;
#47666=CARTESIAN_POINT ( 'NONE',  ( -56.00000000000000711, 3.800000000000001599, -1.887458608817680794 ) ) ;
#47728=AXIS2_PLACEMENT_3D ( 'NONE', #15630, #50836, #41749 ) ;
#47897=VERTEX_POINT ( 'NONE', #47164 ) ;
#47935=EDGE_CURVE ( 'NONE', #51315, #20494, #38371, .T. ) ;
#48028=ORIENTED_EDGE ( 'NONE', *, *, #9865, .T. ) ;
#48099=DIRECTION ( 'NONE',  ( -0.000000000000000000, 0.000000000000000000, 1.000000000000000000 ) ) ;
#48227=DIRECTION ( 'NONE',  ( 0.000000000000000000, -0.000000000000000000, 1.000000000000000000 ) ) ;
#48271=COLOUR_RGB ( '', 0.09019608, 0.27058824, 0.51372549) ;
#48273=LINE ( 'NONE', #13398, #50114 ) ;
#48351=DIRECTION ( 'NONE',  ( 0.000000000000000000, -1.000000000000000000, 0.000000000000000000 ) ) ;
#48386=CIRCLE ( 'NONE', #5758, 0.2499999999999997780 ) ;
#48622=CARTESIAN_POINT ( 'NONE',  ( -56.00000000000000711, 3.800000000000001599, -1.887458608817680794 ) ) ;
#48644=ORIENTED_EDGE ( 'NONE', *, *, #5423, .F. ) ;
#48753=ADVANCED_FACE ( 'NONE', ( #4239 ), #51367, .F. ) ;
#48789=VERTEX_POINT ( 'NONE', #47666 ) ;
#48807=EDGE_CURVE ( 'NONE', #20913, #48789, #5852, .T. ) ;
#49640=ADVANCED_BREP_SHAPE_REPRESENTATION ( '', ( #2411, #2610 ), #38910 ) ;
#49665=CARTESIAN_POINT ( 'NONE',  ( -58.00000000000000711, -9.000000000000000000, 7.102951435054649637E-15 ) ) ;
#49795=CARTESIAN_POINT ( 'NONE',  ( -56.56281744964225311, 4.044141780346881099, 2.346371251900079447 ) ) ;
#50114=VECTOR ( 'NONE', #5155, 1000.000000000000000 ) ;
#50145=ORIENTED_EDGE ( 'NONE', *, *, #21847, .F. ) ;
#50163=B_SPLINE_CURVE_WITH_KNOTS ( 'NONE', 3,
 ( #2848, #20178, #41221, #19352, #6579, #37515, #54006, #14829, #32979, #28156, #24195, #37227, #41511, #36691 ),
 .UNSPECIFIED., .F., .F.,
 ( 4, 2, 2, 2, 2, 2, 4 ),
 ( 2.976959356410394185E-17, 0.0005795730796964416141, 0.001159146159392853304, 0.001448932699241052427, 0.001738719239089251550, 0.002028505778937450890, 0.002318292318785650230 ),
 .UNSPECIFIED. ) ;
#50314=CARTESIAN_POINT ( 'NONE',  ( -58.00000000000000711, -9.250000000000000000, 7.102951435054649637E-15 ) ) ;
#50607=FACE_OUTER_BOUND ( 'NONE', #24686, .T. ) ;
#50717=VERTEX_POINT ( 'NONE', #42147 ) ;
#50836=DIRECTION ( 'NONE',  ( 0.000000000000000000, -1.000000000000000000, 0.000000000000000000 ) ) ;
#50960=FACE_BOUND ( 'NONE', #22431, .T. ) ;
#50984=( GEOMETRIC_REPRESENTATION_CONTEXT ( 3 ) GLOBAL_UNCERTAINTY_ASSIGNED_CONTEXT ( ( #37092 ) ) GLOBAL_UNIT_ASSIGNED_CONTEXT ( ( #3551, #3278, #29396 ) ) REPRESENTATION_CONTEXT ( 'NONE', 'WORKASPACE' ) );
#50989=DIRECTION ( 'NONE',  ( -0.000000000000000000, 1.000000000000000000, -0.000000000000000000 ) ) ;
#51006=VECTOR ( 'NONE', #8786, 1000.000000000000000 ) ;
#51121=SURFACE_SIDE_STYLE ('',( #16474 ) ) ;
#51263=UNCERTAINTY_MEASURE_WITH_UNIT (LENGTH_MEASURE( 1.000000000000000082E-05 ), #26396, 'distance_accuracy_value', 'NONE');
#51315=VERTEX_POINT ( 'NONE', #9965 ) ;
#51317=CARTESIAN_POINT ( 'NONE',  ( -58.00000000000000711, -9.000000000000000000, 7.102951435054649637E-15 ) ) ;
#51346=CARTESIAN_POINT ( 'NONE',  ( -55.98099385706747455, 6.802457008950081097, -1.869625304823616219 ) ) ;
#51367=CYLINDRICAL_SURFACE ( 'NONE', #36608, 0.7500000000000006661 ) ;
#51820=DIRECTION ( 'NONE',  ( 0.000000000000000000, 0.000000000000000000, -1.000000000000000000 ) ) ;
#51821=CARTESIAN_POINT ( 'NONE',  ( -56.75000000000000711, 4.550000000000001599, -2.749999999999994671 ) ) ;
#51905=AXIS2_PLACEMENT_3D ( 'NONE', #10855, #19364, #14559 ) ;
#51973=DIRECTION ( 'NONE',  ( 0.000000000000000000, 0.000000000000000000, -1.000000000000000000 ) ) ;
#52097=CARTESIAN_POINT ( 'NONE',  ( -58.00000000000000711, -9.000000000000000000, 3.457106781186559896 ) ) ;
#52110=FACE_OUTER_BOUND ( 'NONE', #46014, .T. ) ;
#52251=ORIENTED_EDGE ( 'NONE', *, *, #9865, .F. ) ;
#52518=( GEOMETRIC_REPRESENTATION_CONTEXT ( 3 ) GLOBAL_UNCERTAINTY_ASSIGNED_CONTEXT ( ( #55806 ) ) GLOBAL_UNIT_ASSIGNED_CONTEXT ( ( #55666, #25865, #29573 ) ) REPRESENTATION_CONTEXT ( 'NONE', 'WORKASPACE' ) );
#52656=CARTESIAN_POINT ( 'NONE',  ( -58.00000000000000711, -8.999999999999998224, 7.102951435054649637E-15 ) ) ;
#52851=ORIENTED_EDGE ( 'NONE', *, *, #35348, .T. ) ;
#52868=EDGE_LOOP ( 'NONE', ( #40191, #8210, #11689, #8264 ) ) ;
#52950=DIRECTION ( 'NONE',  ( 0.000000000000000000, 1.000000000000000000, 0.000000000000000000 ) ) ;
#53169=CARTESIAN_POINT ( 'NONE',  ( -56.72379438140767149, 4.325189740742904299, -2.436530593025232783 ) ) ;
#53183=EDGE_LOOP ( 'NONE', ( #43475, #34534, #44735, #52251 ) ) ;
#53488=CARTESIAN_POINT ( 'NONE',  ( -56.75000000000000711, 0.000000000000000000, -2.749999999999994671 ) ) ;
#53721=PLANE ( 'NONE',  #51905 ) ;
#54006=CARTESIAN_POINT ( 'NONE',  ( -56.26331385538585295, 6.756938025167550599, 2.134183571387440637 ) ) ;
#54068=AXIS2_PLACEMENT_3D ( 'NONE', #53488, #10333, #48099 ) ;
#54151=AXIS2_PLACEMENT_3D ( 'NONE', #20049, #50989, #15804 ) ;
#54166=DIRECTION ( 'NONE',  ( 0.000000000000000000, -1.000000000000000000, 0.000000000000000000 ) ) ;
#54327=CARTESIAN_POINT ( 'NONE',  ( -56.75000000000000711, 4.550000000000001599, 2.449489742783185875 ) ) ;
#54488=ORIENTED_EDGE ( 'NONE', *, *, #48807, .T. ) ;
#54634=ORIENTED_EDGE ( 'NONE', *, *, #10925, .T. ) ;
#54737=ORIENTED_EDGE ( 'NONE', *, *, #24419, .T. ) ;
#54960=VECTOR ( 'NONE', #13893, 1000.000000000000000 ) ;
#55038=CIRCLE ( 'NONE', #54151, 3.457106781186553235 ) ;
#55068=CARTESIAN_POINT ( 'NONE',  ( -58.00000000000000711, -9.000000000000000000, -2.749999999999994671 ) ) ;
#55238=CARTESIAN_POINT ( 'NONE',  ( -58.00000000000000711, -9.999999999999998224, 2.750000000000013323 ) ) ;
#55252=ORIENTED_EDGE ( 'NONE', *, *, #21847, .T. ) ;
#55322=CARTESIAN_POINT ( 'NONE',  ( -56.00000000000000711, 6.050000000000001599, -2.749999999999994671 ) ) ;
#55389=SHAPE_REPRESENTATION ( 'Swivel Catch Post', ( #2610 ), #38910 ) ;
#55426=LINE ( 'NONE', #11982, #26610 ) ;
#55583=CARTESIAN_POINT ( 'NONE',  ( -56.04969639603970677, 6.801751789163780870, -1.941170806325171139 ) ) ;
#55630=DIRECTION ( 'NONE',  ( 0.000000000000000000, 0.000000000000000000, -1.000000000000000000 ) ) ;
#55666=( LENGTH_UNIT ( ) NAMED_UNIT ( * ) SI_UNIT ( .MILLI., .METRE. ) );
#55718=PLANE ( 'NONE',  #35660 ) ;
#55806=UNCERTAINTY_MEASURE_WITH_UNIT (LENGTH_MEASURE( 1.000000000000000082E-05 ), #55666, 'distance_accuracy_value', 'NONE');
#55979=TOROIDAL_SURFACE ( 'NONE', #6098, 2.750000000000006217, 1.000000000000000000 ) ;
#56017=CIRCLE ( 'NONE', #12488, 2.750000000000006217 ) ;
#56060=FACE_OUTER_BOUND ( 'NONE', #30183, .T. ) ;
#56083=ORIENTED_EDGE ( 'NONE', *, *, #36953, .F. ) ;
#56227=FILL_AREA_STYLE_COLOUR ( '', #16235 ) ;
ENDSEC;
END-ISO-10303-21;
